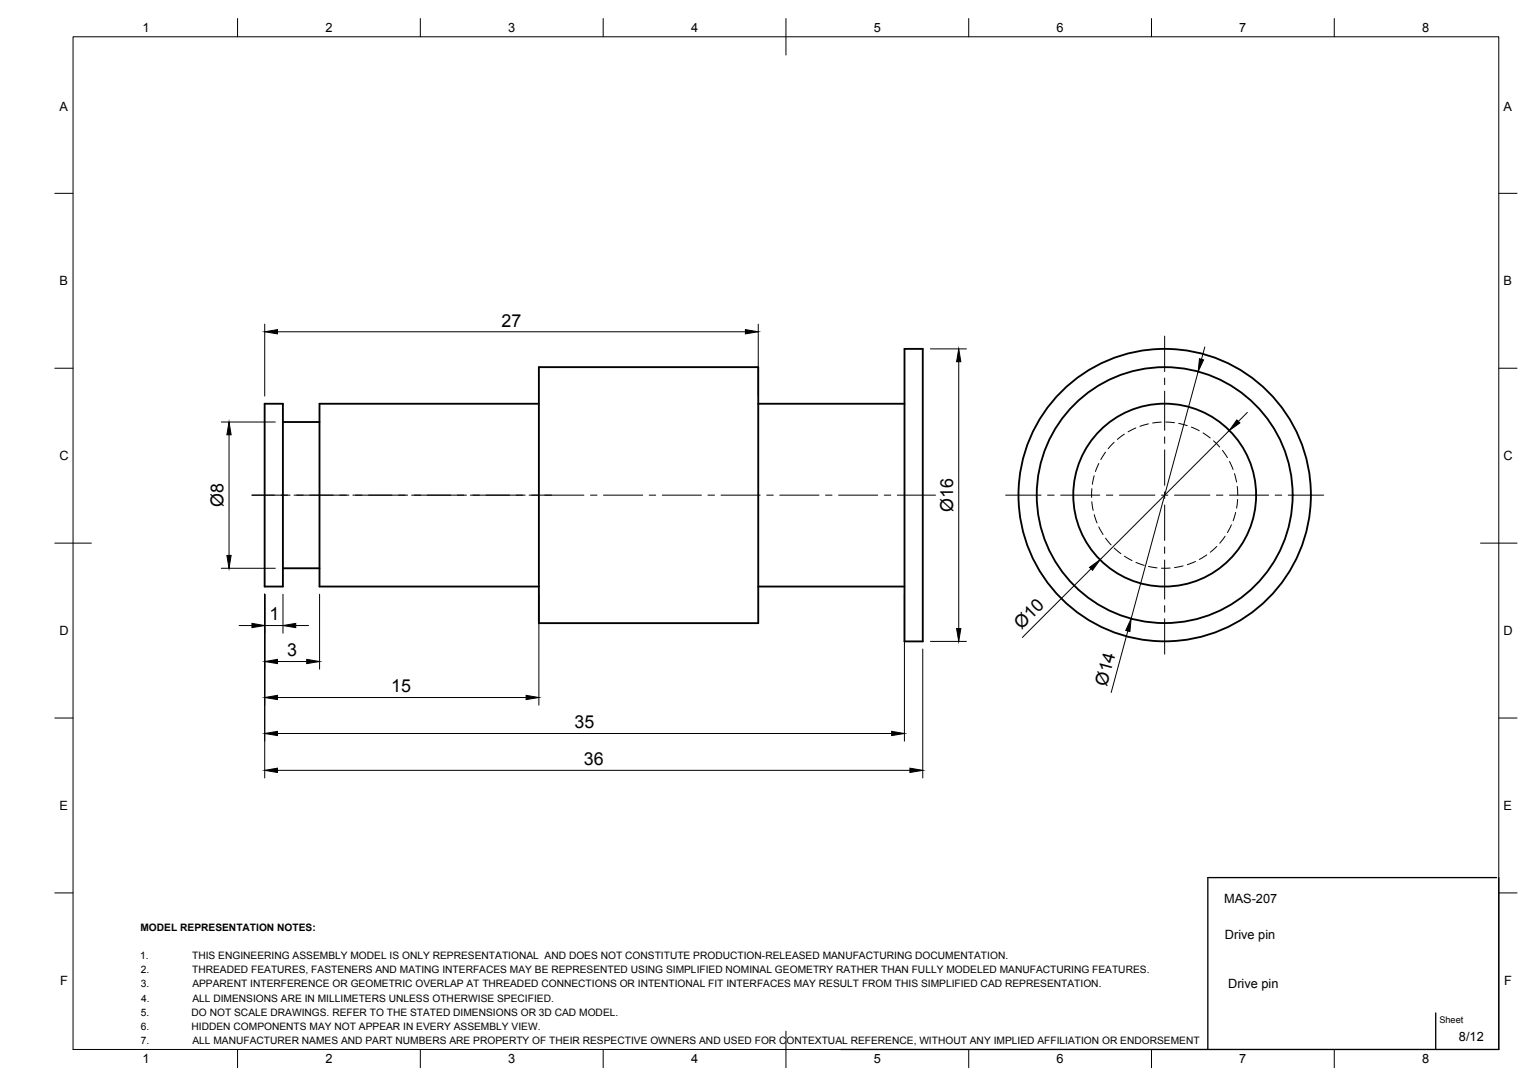
ISO-10303-21;
HEADER;
/* Generated by software containing ST-Developer
 * from STEP Tools, Inc. (www.steptools.com) 
 */

FILE_DESCRIPTION(
/* description */ ('Independent six-slot Geneva indexer. Center distance100, drive radius
50, 60degree indexing per input revolution with120degree engagement an
d240degree dwell. Native machined concave locking faces and relieved d
isk; replaceable retained drive pin; keyed output shaft. Geometry traj
ectory checks use calculated indexing positions, not a contact-dynamic
s simulation. No load or production rating assigned.'),
/* implementation_level */ '2;1');

FILE_NAME(
/* name */ 'Drive pin.step',
/* time_stamp */ '2026-11-09T17:53:22-08:00',
/* author */ (''),
/* organization */ (''),
/* preprocessor_version */ 'ST-DEVELOPER v20.2',
/* originating_system */ 'Autodesk Translation Framework v15.17.0.0',
/* authorisation */ '');

FILE_SCHEMA (('AUTOMOTIVE_DESIGN { 1 0 10303 214 3 1 1 }'));
ENDSEC;

DATA;
#10=MECHANICAL_DESIGN_GEOMETRIC_PRESENTATION_REPRESENTATION('',(#106),#4149);
#84=SHAPE_REPRESENTATION_RELATIONSHIP('SRR','None',#4201,#95);
#95=ADVANCED_BREP_SHAPE_REPRESENTATION('',(#117),#4143);
#106=STYLED_ITEM('',(#4263),#117);
#117=MANIFOLD_SOLID_BREP('Body1',#2300);
#148=FACE_BOUND('',#501,.T.);
#149=FACE_BOUND('',#503,.T.);
#150=FACE_BOUND('',#508,.T.);
#151=FACE_BOUND('',#510,.T.);
#152=FACE_BOUND('',#513,.T.);
#219=PLANE('',#2628);
#220=PLANE('',#2631);
#221=PLANE('',#2640);
#222=PLANE('',#2642);
#223=PLANE('',#2646);
#224=PLANE('',#2650);
#225=PLANE('',#2652);
#339=FACE_OUTER_BOUND('',#500,.T.);
#340=FACE_OUTER_BOUND('',#502,.T.);
#341=FACE_OUTER_BOUND('',#504,.T.);
#342=FACE_OUTER_BOUND('',#505,.T.);
#343=FACE_OUTER_BOUND('',#506,.T.);
#344=FACE_OUTER_BOUND('',#507,.T.);
#345=FACE_OUTER_BOUND('',#509,.T.);
#346=FACE_OUTER_BOUND('',#511,.T.);
#347=FACE_OUTER_BOUND('',#512,.T.);
#348=FACE_OUTER_BOUND('',#514,.T.);
#349=FACE_OUTER_BOUND('',#515,.T.);
#350=FACE_OUTER_BOUND('',#516,.T.);
#351=FACE_OUTER_BOUND('',#517,.T.);
#500=EDGE_LOOP('',(#1992));
#501=EDGE_LOOP('',(#1993));
#502=EDGE_LOOP('',(#1994));
#503=EDGE_LOOP('',(#1995));
#504=EDGE_LOOP('',(#1996,#1997,#1998,#1999));
#505=EDGE_LOOP('',(#2000,#2001,#2002,#2003));
#506=EDGE_LOOP('',(#2004,#2005,#2006,#2007));
#507=EDGE_LOOP('',(#2008));
#508=EDGE_LOOP('',(#2009));
#509=EDGE_LOOP('',(#2010));
#510=EDGE_LOOP('',(#2011));
#511=EDGE_LOOP('',(#2012,#2013,#2014,#2015));
#512=EDGE_LOOP('',(#2016));
#513=EDGE_LOOP('',(#2017));
#514=EDGE_LOOP('',(#2018,#2019,#2020,#2021));
#515=EDGE_LOOP('',(#2022));
#516=EDGE_LOOP('',(#2023,#2024,#2025,#2026));
#517=EDGE_LOOP('',(#2027));
#698=LINE('',#3988,#870);
#699=LINE('',#3991,#871);
#700=LINE('',#3997,#872);
#701=LINE('',#4008,#873);
#702=LINE('',#4014,#874);
#703=LINE('',#4018,#875);
#870=VECTOR('',#3281,7.);
#871=VECTOR('',#3284,5.);
#872=VECTOR('',#3291,4.);
#873=VECTOR('',#3306,5.);
#874=VECTOR('',#3313,8.);
#875=VECTOR('',#3320,5.);
#984=CIRCLE('',#2629,7.);
#985=CIRCLE('',#2630,5.);
#986=CIRCLE('',#2632,7.);
#987=CIRCLE('',#2633,5.);
#988=CIRCLE('',#2636,5.);
#989=CIRCLE('',#2638,4.);
#990=CIRCLE('',#2639,4.);
#991=CIRCLE('',#2641,5.);
#992=CIRCLE('',#2643,5.);
#993=CIRCLE('',#2645,5.);
#994=CIRCLE('',#2647,8.);
#995=CIRCLE('',#2649,8.);
#1176=VERTEX_POINT('',#3978);
#1177=VERTEX_POINT('',#3980);
#1178=VERTEX_POINT('',#3983);
#1179=VERTEX_POINT('',#3985);
#1180=VERTEX_POINT('',#3990);
#1181=VERTEX_POINT('',#3994);
#1182=VERTEX_POINT('',#3996);
#1183=VERTEX_POINT('',#4000);
#1184=VERTEX_POINT('',#4003);
#1185=VERTEX_POINT('',#4006);
#1186=VERTEX_POINT('',#4010);
#1187=VERTEX_POINT('',#4013);
#1454=EDGE_CURVE('',#1176,#1176,#984,.T.);
#1455=EDGE_CURVE('',#1177,#1177,#985,.T.);
#1456=EDGE_CURVE('',#1178,#1178,#986,.T.);
#1457=EDGE_CURVE('',#1179,#1179,#987,.T.);
#1458=EDGE_CURVE('',#1176,#1178,#698,.T.);
#1459=EDGE_CURVE('',#1179,#1180,#699,.T.);
#1460=EDGE_CURVE('',#1180,#1180,#988,.T.);
#1461=EDGE_CURVE('',#1181,#1181,#989,.T.);
#1462=EDGE_CURVE('',#1181,#1182,#700,.T.);
#1463=EDGE_CURVE('',#1182,#1182,#990,.T.);
#1464=EDGE_CURVE('',#1183,#1183,#991,.T.);
#1465=EDGE_CURVE('',#1184,#1184,#992,.T.);
#1466=EDGE_CURVE('',#1185,#1185,#993,.T.);
#1467=EDGE_CURVE('',#1185,#1184,#701,.T.);
#1468=EDGE_CURVE('',#1186,#1186,#994,.T.);
#1469=EDGE_CURVE('',#1186,#1187,#702,.T.);
#1470=EDGE_CURVE('',#1187,#1187,#995,.T.);
#1471=EDGE_CURVE('',#1183,#1177,#703,.T.);
#1992=ORIENTED_EDGE('',*,*,#1454,.T.);
#1993=ORIENTED_EDGE('',*,*,#1455,.F.);
#1994=ORIENTED_EDGE('',*,*,#1456,.F.);
#1995=ORIENTED_EDGE('',*,*,#1457,.F.);
#1996=ORIENTED_EDGE('',*,*,#1454,.F.);
#1997=ORIENTED_EDGE('',*,*,#1458,.T.);
#1998=ORIENTED_EDGE('',*,*,#1456,.T.);
#1999=ORIENTED_EDGE('',*,*,#1458,.F.);
#2000=ORIENTED_EDGE('',*,*,#1457,.T.);
#2001=ORIENTED_EDGE('',*,*,#1459,.T.);
#2002=ORIENTED_EDGE('',*,*,#1460,.T.);
#2003=ORIENTED_EDGE('',*,*,#1459,.F.);
#2004=ORIENTED_EDGE('',*,*,#1461,.T.);
#2005=ORIENTED_EDGE('',*,*,#1462,.T.);
#2006=ORIENTED_EDGE('',*,*,#1463,.F.);
#2007=ORIENTED_EDGE('',*,*,#1462,.F.);
#2008=ORIENTED_EDGE('',*,*,#1464,.F.);
#2009=ORIENTED_EDGE('',*,*,#1461,.F.);
#2010=ORIENTED_EDGE('',*,*,#1465,.F.);
#2011=ORIENTED_EDGE('',*,*,#1463,.T.);
#2012=ORIENTED_EDGE('',*,*,#1466,.F.);
#2013=ORIENTED_EDGE('',*,*,#1467,.T.);
#2014=ORIENTED_EDGE('',*,*,#1465,.T.);
#2015=ORIENTED_EDGE('',*,*,#1467,.F.);
#2016=ORIENTED_EDGE('',*,*,#1468,.T.);
#2017=ORIENTED_EDGE('',*,*,#1460,.F.);
#2018=ORIENTED_EDGE('',*,*,#1468,.F.);
#2019=ORIENTED_EDGE('',*,*,#1469,.T.);
#2020=ORIENTED_EDGE('',*,*,#1470,.T.);
#2021=ORIENTED_EDGE('',*,*,#1469,.F.);
#2022=ORIENTED_EDGE('',*,*,#1470,.F.);
#2023=ORIENTED_EDGE('',*,*,#1464,.T.);
#2024=ORIENTED_EDGE('',*,*,#1471,.T.);
#2025=ORIENTED_EDGE('',*,*,#1455,.T.);
#2026=ORIENTED_EDGE('',*,*,#1471,.F.);
#2027=ORIENTED_EDGE('',*,*,#1466,.T.);
#2143=CYLINDRICAL_SURFACE('',#2634,7.);
#2144=CYLINDRICAL_SURFACE('',#2635,5.);
#2145=CYLINDRICAL_SURFACE('',#2637,4.);
#2146=CYLINDRICAL_SURFACE('',#2644,5.);
#2147=CYLINDRICAL_SURFACE('',#2648,8.);
#2148=CYLINDRICAL_SURFACE('',#2651,5.);
#2260=ADVANCED_FACE('',(#339,#148),#219,.T.);
#2261=ADVANCED_FACE('',(#340,#149),#220,.F.);
#2262=ADVANCED_FACE('',(#341),#2143,.T.);
#2263=ADVANCED_FACE('',(#342),#2144,.T.);
#2264=ADVANCED_FACE('',(#343),#2145,.T.);
#2265=ADVANCED_FACE('',(#344,#150),#221,.F.);
#2266=ADVANCED_FACE('',(#345,#151),#222,.F.);
#2267=ADVANCED_FACE('',(#346),#2146,.T.);
#2268=ADVANCED_FACE('',(#347,#152),#223,.T.);
#2269=ADVANCED_FACE('',(#348),#2147,.T.);
#2270=ADVANCED_FACE('',(#349),#224,.F.);
#2271=ADVANCED_FACE('',(#350),#2148,.T.);
#2272=ADVANCED_FACE('',(#351),#225,.T.);
#2300=CLOSED_SHELL('',(#2260,#2261,#2262,#2263,#2264,#2265,#2266,#2267,
#2268,#2269,#2270,#2271,#2272));
#2627=AXIS2_PLACEMENT_3D('',#3976,#3265,#3266);
#2628=AXIS2_PLACEMENT_3D('',#3977,#3267,#3268);
#2629=AXIS2_PLACEMENT_3D('',#3979,#3269,#3270);
#2630=AXIS2_PLACEMENT_3D('',#3981,#3271,#3272);
#2631=AXIS2_PLACEMENT_3D('',#3982,#3273,#3274);
#2632=AXIS2_PLACEMENT_3D('',#3984,#3275,#3276);
#2633=AXIS2_PLACEMENT_3D('',#3986,#3277,#3278);
#2634=AXIS2_PLACEMENT_3D('',#3987,#3279,#3280);
#2635=AXIS2_PLACEMENT_3D('',#3989,#3282,#3283);
#2636=AXIS2_PLACEMENT_3D('',#3992,#3285,#3286);
#2637=AXIS2_PLACEMENT_3D('',#3993,#3287,#3288);
#2638=AXIS2_PLACEMENT_3D('',#3995,#3289,#3290);
#2639=AXIS2_PLACEMENT_3D('',#3998,#3292,#3293);
#2640=AXIS2_PLACEMENT_3D('',#3999,#3294,#3295);
#2641=AXIS2_PLACEMENT_3D('',#4001,#3296,#3297);
#2642=AXIS2_PLACEMENT_3D('',#4002,#3298,#3299);
#2643=AXIS2_PLACEMENT_3D('',#4004,#3300,#3301);
#2644=AXIS2_PLACEMENT_3D('',#4005,#3302,#3303);
#2645=AXIS2_PLACEMENT_3D('',#4007,#3304,#3305);
#2646=AXIS2_PLACEMENT_3D('',#4009,#3307,#3308);
#2647=AXIS2_PLACEMENT_3D('',#4011,#3309,#3310);
#2648=AXIS2_PLACEMENT_3D('',#4012,#3311,#3312);
#2649=AXIS2_PLACEMENT_3D('',#4015,#3314,#3315);
#2650=AXIS2_PLACEMENT_3D('',#4016,#3316,#3317);
#2651=AXIS2_PLACEMENT_3D('',#4017,#3318,#3319);
#2652=AXIS2_PLACEMENT_3D('',#4019,#3321,#3322);
#3265=DIRECTION('axis',(0.,0.,1.));
#3266=DIRECTION('refdir',(1.,0.,0.));
#3267=DIRECTION('center_axis',(0.,0.,1.));
#3268=DIRECTION('ref_axis',(1.,0.,0.));
#3269=DIRECTION('center_axis',(0.,0.,1.));
#3270=DIRECTION('ref_axis',(1.,0.,0.));
#3271=DIRECTION('center_axis',(0.,0.,1.));
#3272=DIRECTION('ref_axis',(1.,0.,0.));
#3273=DIRECTION('center_axis',(0.,0.,1.));
#3274=DIRECTION('ref_axis',(1.,0.,0.));
#3275=DIRECTION('center_axis',(0.,0.,1.));
#3276=DIRECTION('ref_axis',(1.,0.,0.));
#3277=DIRECTION('center_axis',(0.,0.,-1.));
#3278=DIRECTION('ref_axis',(1.,0.,0.));
#3279=DIRECTION('center_axis',(0.,0.,1.));
#3280=DIRECTION('ref_axis',(1.,0.,0.));
#3281=DIRECTION('',(0.,0.,-1.));
#3282=DIRECTION('center_axis',(0.,0.,1.));
#3283=DIRECTION('ref_axis',(1.,0.,0.));
#3284=DIRECTION('',(0.,0.,-1.));
#3285=DIRECTION('center_axis',(0.,0.,1.));
#3286=DIRECTION('ref_axis',(1.,0.,0.));
#3287=DIRECTION('center_axis',(0.,0.,1.));
#3288=DIRECTION('ref_axis',(1.,0.,0.));
#3289=DIRECTION('center_axis',(0.,0.,1.));
#3290=DIRECTION('ref_axis',(1.,0.,0.));
#3291=DIRECTION('',(0.,0.,1.));
#3292=DIRECTION('center_axis',(0.,0.,1.));
#3293=DIRECTION('ref_axis',(1.,0.,0.));
#3294=DIRECTION('center_axis',(0.,0.,-1.));
#3295=DIRECTION('ref_axis',(-1.,0.,0.));
#3296=DIRECTION('center_axis',(0.,0.,-1.));
#3297=DIRECTION('ref_axis',(1.,0.,0.));
#3298=DIRECTION('center_axis',(0.,0.,1.));
#3299=DIRECTION('ref_axis',(1.,0.,0.));
#3300=DIRECTION('center_axis',(0.,0.,1.));
#3301=DIRECTION('ref_axis',(1.,0.,0.));
#3302=DIRECTION('center_axis',(0.,0.,1.));
#3303=DIRECTION('ref_axis',(1.,0.,0.));
#3304=DIRECTION('center_axis',(0.,0.,1.));
#3305=DIRECTION('ref_axis',(1.,0.,0.));
#3306=DIRECTION('',(0.,0.,-1.));
#3307=DIRECTION('center_axis',(0.,0.,1.));
#3308=DIRECTION('ref_axis',(1.,0.,0.));
#3309=DIRECTION('center_axis',(0.,0.,1.));
#3310=DIRECTION('ref_axis',(1.,0.,0.));
#3311=DIRECTION('center_axis',(0.,0.,1.));
#3312=DIRECTION('ref_axis',(1.,0.,0.));
#3313=DIRECTION('',(0.,0.,-1.));
#3314=DIRECTION('center_axis',(0.,0.,1.));
#3315=DIRECTION('ref_axis',(1.,0.,0.));
#3316=DIRECTION('center_axis',(0.,0.,1.));
#3317=DIRECTION('ref_axis',(1.,0.,0.));
#3318=DIRECTION('center_axis',(0.,0.,1.));
#3319=DIRECTION('ref_axis',(1.,0.,0.));
#3320=DIRECTION('',(0.,0.,-1.));
#3321=DIRECTION('center_axis',(0.,0.,1.));
#3322=DIRECTION('ref_axis',(1.,0.,0.));
#3976=CARTESIAN_POINT('',(0.,0.,0.));
#3977=CARTESIAN_POINT('Origin',(0.,0.,20.));
#3978=CARTESIAN_POINT('',(-7.,-8.57252759403147E-16,20.));
#3979=CARTESIAN_POINT('Origin',(0.,0.,20.));
#3980=CARTESIAN_POINT('',(-5.,-6.12323399573677E-16,20.));
#3981=CARTESIAN_POINT('Origin',(0.,0.,20.));
#3982=CARTESIAN_POINT('Origin',(0.,0.,8.));
#3983=CARTESIAN_POINT('',(-7.,-8.57252759403147E-16,8.));
#3984=CARTESIAN_POINT('Origin',(0.,0.,8.));
#3985=CARTESIAN_POINT('',(-5.,6.12323399573677E-16,8.));
#3986=CARTESIAN_POINT('Origin',(0.,0.,8.));
#3987=CARTESIAN_POINT('Origin',(0.,0.,8.));
#3988=CARTESIAN_POINT('',(-7.,-8.57252759403147E-16,8.));
#3989=CARTESIAN_POINT('Origin',(0.,0.,0.));
#3990=CARTESIAN_POINT('',(-5.,-6.12323399573677E-16,0.));
#3991=CARTESIAN_POINT('',(-5.,-6.12323399573677E-16,0.));
#3992=CARTESIAN_POINT('Origin',(0.,0.,0.));
#3993=CARTESIAN_POINT('Origin',(0.,0.,33.));
#3994=CARTESIAN_POINT('',(-4.,-4.89858719658941E-16,32.));
#3995=CARTESIAN_POINT('Origin',(0.,0.,32.));
#3996=CARTESIAN_POINT('',(-4.,-4.89858719658941E-16,34.));
#3997=CARTESIAN_POINT('',(-4.,-4.89858719658941E-16,33.));
#3998=CARTESIAN_POINT('Origin',(0.,0.,34.));
#3999=CARTESIAN_POINT('Origin',(8.,0.,32.));
#4000=CARTESIAN_POINT('',(-5.,6.12323399573677E-16,32.));
#4001=CARTESIAN_POINT('Origin',(0.,0.,32.));
#4002=CARTESIAN_POINT('Origin',(4.,0.,34.));
#4003=CARTESIAN_POINT('',(-5.,-6.12323399573677E-16,34.));
#4004=CARTESIAN_POINT('Origin',(0.,0.,34.));
#4005=CARTESIAN_POINT('Origin',(0.,0.,0.));
#4006=CARTESIAN_POINT('',(-5.,-6.12323399573677E-16,35.));
#4007=CARTESIAN_POINT('Origin',(0.,0.,35.));
#4008=CARTESIAN_POINT('',(-5.,-6.12323399573677E-16,0.));
#4009=CARTESIAN_POINT('Origin',(0.,0.,0.));
#4010=CARTESIAN_POINT('',(-8.,-9.79717439317883E-16,0.));
#4011=CARTESIAN_POINT('Origin',(0.,0.,0.));
#4012=CARTESIAN_POINT('Origin',(0.,0.,-1.));
#4013=CARTESIAN_POINT('',(-8.,-9.79717439317883E-16,-1.));
#4014=CARTESIAN_POINT('',(-8.,-9.79717439317883E-16,-1.));
#4015=CARTESIAN_POINT('Origin',(0.,0.,-1.));
#4016=CARTESIAN_POINT('Origin',(0.,0.,-1.));
#4017=CARTESIAN_POINT('Origin',(0.,0.,0.));
#4018=CARTESIAN_POINT('',(-5.,-6.12323399573677E-16,0.));
#4019=CARTESIAN_POINT('Origin',(0.,0.,35.));
#4130=UNCERTAINTY_MEASURE_WITH_UNIT(LENGTH_MEASURE(0.01),#4150,
'DISTANCE_ACCURACY_VALUE',
'Maximum model space distance between geometric entities at asserted c
onnectivities');
#4136=UNCERTAINTY_MEASURE_WITH_UNIT(LENGTH_MEASURE(0.01),#4150,
'DISTANCE_ACCURACY_VALUE',
'Maximum model space distance between geometric entities at asserted c
onnectivities');
#4143=(
GEOMETRIC_REPRESENTATION_CONTEXT(3)
GLOBAL_UNCERTAINTY_ASSIGNED_CONTEXT((#4130))
GLOBAL_UNIT_ASSIGNED_CONTEXT((#4150,#4152,#4153))
REPRESENTATION_CONTEXT('','3D')
);
#4149=(
GEOMETRIC_REPRESENTATION_CONTEXT(3)
GLOBAL_UNCERTAINTY_ASSIGNED_CONTEXT((#4136))
GLOBAL_UNIT_ASSIGNED_CONTEXT((#4150,#4152,#4153))
REPRESENTATION_CONTEXT('','3D')
);
#4150=(
LENGTH_UNIT()
NAMED_UNIT(*)
SI_UNIT(.MILLI.,.METRE.)
);
#4152=(
NAMED_UNIT(*)
PLANE_ANGLE_UNIT()
SI_UNIT($,.RADIAN.)
);
#4153=(
NAMED_UNIT(*)
SI_UNIT($,.STERADIAN.)
SOLID_ANGLE_UNIT()
);
#4160=SHAPE_DEFINITION_REPRESENTATION(#4172,#4201);
#4172=PRODUCT_DEFINITION_SHAPE('',$,#4214);
#4201=SHAPE_REPRESENTATION('',(#2627),#4143);
#4207=PRODUCT_DEFINITION_CONTEXT('part definition',#4245,'design');
#4214=PRODUCT_DEFINITION('Drive pin','Drive pin',#4226,#4207);
#4226=PRODUCT_DEFINITION_FORMATION('',$,#4253);
#4245=APPLICATION_CONTEXT(
'Core Data for Automotive Mechanical Design Process');
#4246=PRODUCT_CONTEXT('part definition',#4245,'mechanical');
#4253=PRODUCT('Drive pin','Drive pin','Drive pin',(#4246));
#4263=PRESENTATION_STYLE_ASSIGNMENT((#4273));
#4273=SURFACE_STYLE_USAGE(.BOTH.,#4283);
#4283=SURFACE_SIDE_STYLE('',(#4293));
#4293=SURFACE_STYLE_FILL_AREA(#4303);
#4303=FILL_AREA_STYLE('Pivot gray',(#4313));
#4313=FILL_AREA_STYLE_COLOUR('Pivot gray',#4323);
#4323=COLOUR_RGB('Pivot gray',0.407843137254902,0.447058823529412,0.498039215686275);
ENDSEC;
END-ISO-10303-21;
